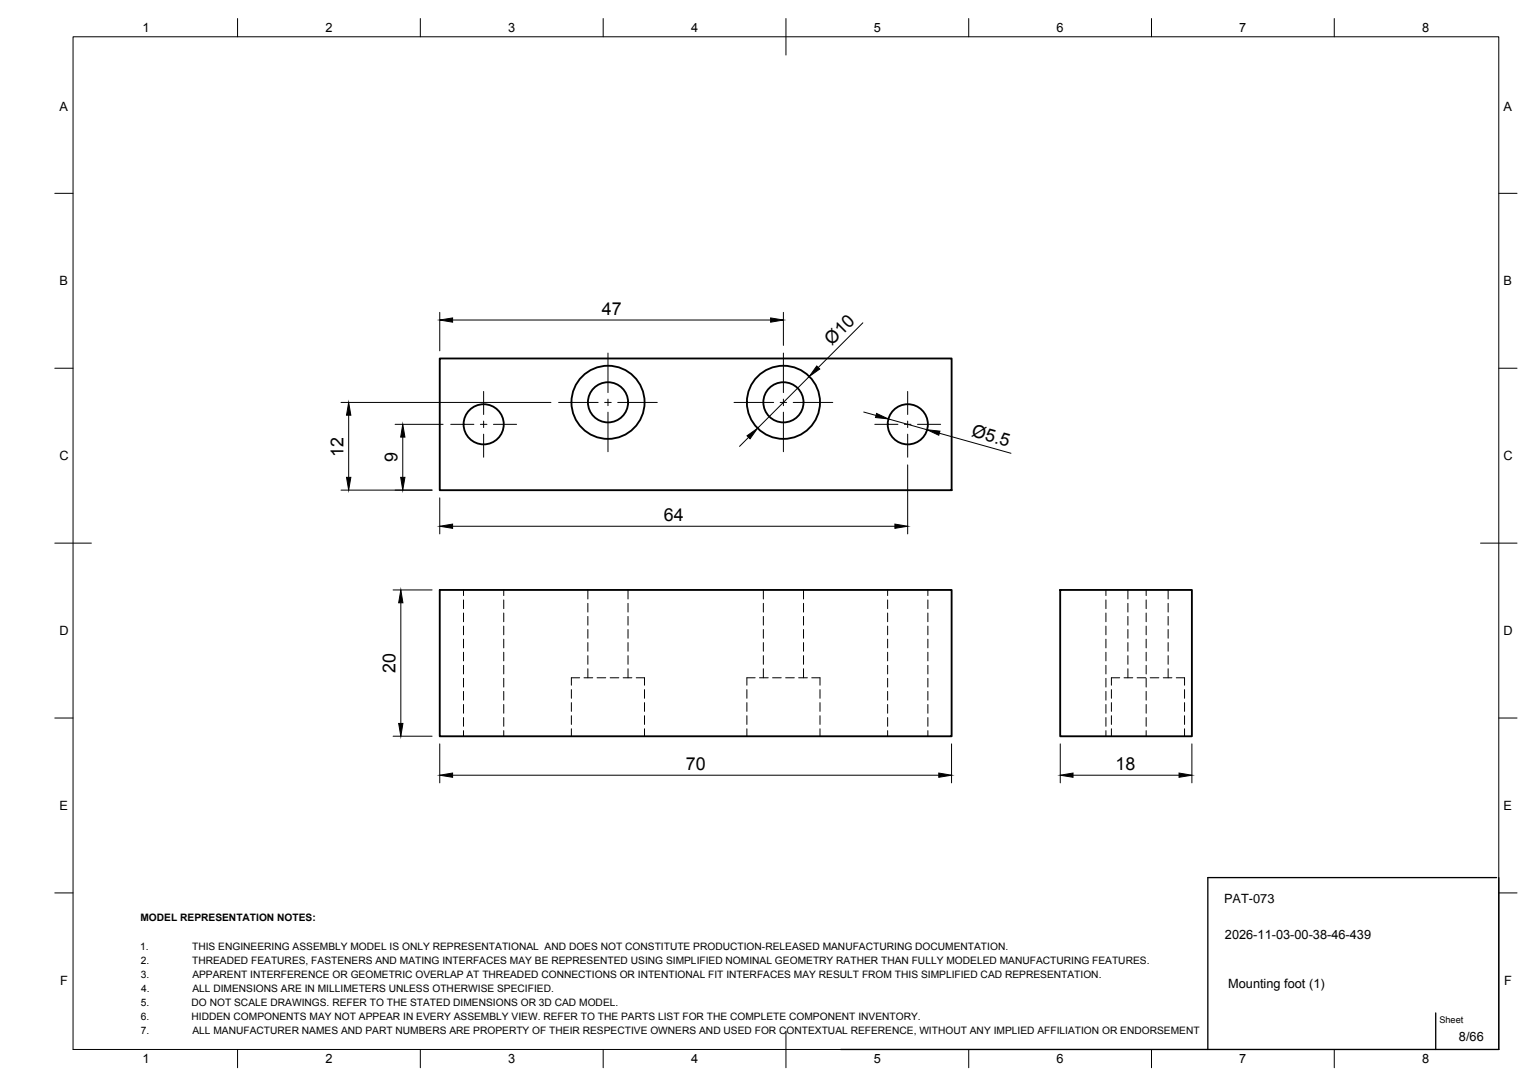
ISO-10303-21;
HEADER;
/* Generated by software containing ST-Developer
 * from STEP Tools, Inc. (www.steptools.com) 
 */

FILE_DESCRIPTION(
/* description */ ('Manual piston pump'),
/* implementation_level */ '2;1');

FILE_NAME(
/* name */ 'Mounting foot (1).step',
/* time_stamp */ '2026-11-02T16:54:23-08:00',
/* author */ (''),
/* organization */ (''),
/* preprocessor_version */ 'ST-DEVELOPER v20.2',
/* originating_system */ 'Autodesk Translation Framework v15.17.0.0',
/* authorisation */ '');

FILE_SCHEMA (('AUTOMOTIVE_DESIGN { 1 0 10303 214 3 1 1 }'));
ENDSEC;

DATA;
#10=MECHANICAL_DESIGN_GEOMETRIC_PRESENTATION_REPRESENTATION('',(#691),#19043);
#565=SHAPE_REPRESENTATION_RELATIONSHIP('SRR','None',#19311,#628);
#628=ADVANCED_BREP_SHAPE_REPRESENTATION('',(#763),#18978);
#691=STYLED_ITEM('',(#19662),#763);
#763=MANIFOLD_SOLID_BREP('Body1',#9475);
#864=FACE_BOUND('',#1974,.T.);
#865=FACE_BOUND('',#1977,.T.);
#866=FACE_BOUND('',#1985,.T.);
#867=FACE_BOUND('',#1986,.T.);
#868=FACE_BOUND('',#1987,.T.);
#869=FACE_BOUND('',#1988,.T.);
#870=FACE_BOUND('',#1990,.T.);
#871=FACE_BOUND('',#1991,.T.);
#872=FACE_BOUND('',#1992,.T.);
#873=FACE_BOUND('',#1993,.T.);
#1122=CYLINDRICAL_SURFACE('',#10379,0.275);
#1123=CYLINDRICAL_SURFACE('',#10382,0.275);
#1124=CYLINDRICAL_SURFACE('',#10385,0.5);
#1125=CYLINDRICAL_SURFACE('',#10390,0.5);
#1126=CYLINDRICAL_SURFACE('',#10395,0.275);
#1127=CYLINDRICAL_SURFACE('',#10397,0.275);
#1358=FACE_OUTER_BOUND('',#1970,.T.);
#1359=FACE_OUTER_BOUND('',#1971,.T.);
#1360=FACE_OUTER_BOUND('',#1972,.T.);
#1361=FACE_OUTER_BOUND('',#1973,.T.);
#1362=FACE_OUTER_BOUND('',#1975,.T.);
#1363=FACE_OUTER_BOUND('',#1976,.T.);
#1364=FACE_OUTER_BOUND('',#1978,.T.);
#1365=FACE_OUTER_BOUND('',#1979,.T.);
#1366=FACE_OUTER_BOUND('',#1980,.T.);
#1367=FACE_OUTER_BOUND('',#1981,.T.);
#1368=FACE_OUTER_BOUND('',#1982,.T.);
#1369=FACE_OUTER_BOUND('',#1983,.T.);
#1370=FACE_OUTER_BOUND('',#1984,.T.);
#1371=FACE_OUTER_BOUND('',#1989,.T.);
#1970=EDGE_LOOP('',(#6587,#6588,#6589,#6590));
#1971=EDGE_LOOP('',(#6591,#6592,#6593,#6594));
#1972=EDGE_LOOP('',(#6595,#6596,#6597,#6598));
#1973=EDGE_LOOP('',(#6599));
#1974=EDGE_LOOP('',(#6600));
#1975=EDGE_LOOP('',(#6601,#6602,#6603,#6604));
#1976=EDGE_LOOP('',(#6605));
#1977=EDGE_LOOP('',(#6606));
#1978=EDGE_LOOP('',(#6607,#6608,#6609,#6610));
#1979=EDGE_LOOP('',(#6611,#6612,#6613,#6614));
#1980=EDGE_LOOP('',(#6615,#6616,#6617,#6618));
#1981=EDGE_LOOP('',(#6619,#6620,#6621,#6622));
#1982=EDGE_LOOP('',(#6623,#6624,#6625,#6626));
#1983=EDGE_LOOP('',(#6627,#6628,#6629,#6630));
#1984=EDGE_LOOP('',(#6631,#6632,#6633,#6634));
#1985=EDGE_LOOP('',(#6635));
#1986=EDGE_LOOP('',(#6636));
#1987=EDGE_LOOP('',(#6637));
#1988=EDGE_LOOP('',(#6638));
#1989=EDGE_LOOP('',(#6639,#6640,#6641,#6642));
#1990=EDGE_LOOP('',(#6643));
#1991=EDGE_LOOP('',(#6644));
#1992=EDGE_LOOP('',(#6645));
#1993=EDGE_LOOP('',(#6646));
#2727=CIRCLE('',#10380,0.275);
#2728=CIRCLE('',#10381,0.275);
#2729=CIRCLE('',#10383,0.275);
#2730=CIRCLE('',#10384,0.275);
#2731=CIRCLE('',#10386,0.5);
#2732=CIRCLE('',#10387,0.5);
#2733=CIRCLE('',#10389,0.275);
#2734=CIRCLE('',#10391,0.5);
#2735=CIRCLE('',#10392,0.5);
#2736=CIRCLE('',#10394,0.275);
#2737=CIRCLE('',#10396,0.275);
#2738=CIRCLE('',#10398,0.275);
#3237=LINE('',#14991,#3841);
#3238=LINE('',#14997,#3842);
#3239=LINE('',#15003,#3843);
#3240=LINE('',#15012,#3844);
#3241=LINE('',#15019,#3845);
#3242=LINE('',#15023,#3846);
#3243=LINE('',#15028,#3847);
#3244=LINE('',#15030,#3848);
#3245=LINE('',#15032,#3849);
#3246=LINE('',#15033,#3850);
#3247=LINE('',#15036,#3851);
#3248=LINE('',#15038,#3852);
#3249=LINE('',#15039,#3853);
#3250=LINE('',#15042,#3854);
#3251=LINE('',#15044,#3855);
#3252=LINE('',#15045,#3856);
#3253=LINE('',#15047,#3857);
#3254=LINE('',#15048,#3858);
#3841=VECTOR('',#11861,0.275);
#3842=VECTOR('',#11868,0.275);
#3843=VECTOR('',#11875,0.5);
#3844=VECTOR('',#11886,0.5);
#3845=VECTOR('',#11895,0.275);
#3846=VECTOR('',#11900,0.275);
#3847=VECTOR('',#11905,1.);
#3848=VECTOR('',#11906,1.);
#3849=VECTOR('',#11907,1.);
#3850=VECTOR('',#11908,1.);
#3851=VECTOR('',#11911,1.);
#3852=VECTOR('',#11912,1.);
#3853=VECTOR('',#11913,1.);
#3854=VECTOR('',#11916,1.);
#3855=VECTOR('',#11917,1.);
#3856=VECTOR('',#11918,1.);
#3857=VECTOR('',#11921,1.);
#3858=VECTOR('',#11922,1.);
#4459=VERTEX_POINT('',#14988);
#4460=VERTEX_POINT('',#14990);
#4461=VERTEX_POINT('',#14994);
#4462=VERTEX_POINT('',#14996);
#4463=VERTEX_POINT('',#15000);
#4464=VERTEX_POINT('',#15002);
#4465=VERTEX_POINT('',#15006);
#4466=VERTEX_POINT('',#15009);
#4467=VERTEX_POINT('',#15011);
#4468=VERTEX_POINT('',#15015);
#4469=VERTEX_POINT('',#15018);
#4470=VERTEX_POINT('',#15022);
#4471=VERTEX_POINT('',#15026);
#4472=VERTEX_POINT('',#15027);
#4473=VERTEX_POINT('',#15029);
#4474=VERTEX_POINT('',#15031);
#4475=VERTEX_POINT('',#15035);
#4476=VERTEX_POINT('',#15037);
#4477=VERTEX_POINT('',#15041);
#4478=VERTEX_POINT('',#15043);
#5280=EDGE_CURVE('',#4459,#4459,#2727,.T.);
#5281=EDGE_CURVE('',#4459,#4460,#3237,.T.);
#5282=EDGE_CURVE('',#4460,#4460,#2728,.T.);
#5283=EDGE_CURVE('',#4461,#4461,#2729,.T.);
#5284=EDGE_CURVE('',#4461,#4462,#3238,.T.);
#5285=EDGE_CURVE('',#4462,#4462,#2730,.T.);
#5286=EDGE_CURVE('',#4463,#4463,#2731,.T.);
#5287=EDGE_CURVE('',#4463,#4464,#3239,.T.);
#5288=EDGE_CURVE('',#4464,#4464,#2732,.T.);
#5289=EDGE_CURVE('',#4465,#4465,#2733,.T.);
#5290=EDGE_CURVE('',#4466,#4466,#2734,.T.);
#5291=EDGE_CURVE('',#4466,#4467,#3240,.T.);
#5292=EDGE_CURVE('',#4467,#4467,#2735,.T.);
#5293=EDGE_CURVE('',#4468,#4468,#2736,.T.);
#5294=EDGE_CURVE('',#4465,#4469,#3241,.T.);
#5295=EDGE_CURVE('',#4469,#4469,#2737,.T.);
#5296=EDGE_CURVE('',#4468,#4470,#3242,.T.);
#5297=EDGE_CURVE('',#4470,#4470,#2738,.T.);
#5298=EDGE_CURVE('',#4471,#4472,#3243,.T.);
#5299=EDGE_CURVE('',#4472,#4473,#3244,.T.);
#5300=EDGE_CURVE('',#4474,#4473,#3245,.T.);
#5301=EDGE_CURVE('',#4471,#4474,#3246,.T.);
#5302=EDGE_CURVE('',#4475,#4471,#3247,.T.);
#5303=EDGE_CURVE('',#4476,#4474,#3248,.T.);
#5304=EDGE_CURVE('',#4475,#4476,#3249,.T.);
#5305=EDGE_CURVE('',#4477,#4475,#3250,.T.);
#5306=EDGE_CURVE('',#4478,#4476,#3251,.T.);
#5307=EDGE_CURVE('',#4477,#4478,#3252,.T.);
#5308=EDGE_CURVE('',#4472,#4477,#3253,.T.);
#5309=EDGE_CURVE('',#4473,#4478,#3254,.T.);
#6587=ORIENTED_EDGE('',*,*,#5280,.F.);
#6588=ORIENTED_EDGE('',*,*,#5281,.T.);
#6589=ORIENTED_EDGE('',*,*,#5282,.F.);
#6590=ORIENTED_EDGE('',*,*,#5281,.F.);
#6591=ORIENTED_EDGE('',*,*,#5283,.F.);
#6592=ORIENTED_EDGE('',*,*,#5284,.T.);
#6593=ORIENTED_EDGE('',*,*,#5285,.F.);
#6594=ORIENTED_EDGE('',*,*,#5284,.F.);
#6595=ORIENTED_EDGE('',*,*,#5286,.F.);
#6596=ORIENTED_EDGE('',*,*,#5287,.T.);
#6597=ORIENTED_EDGE('',*,*,#5288,.T.);
#6598=ORIENTED_EDGE('',*,*,#5287,.F.);
#6599=ORIENTED_EDGE('',*,*,#5288,.F.);
#6600=ORIENTED_EDGE('',*,*,#5289,.F.);
#6601=ORIENTED_EDGE('',*,*,#5290,.F.);
#6602=ORIENTED_EDGE('',*,*,#5291,.T.);
#6603=ORIENTED_EDGE('',*,*,#5292,.T.);
#6604=ORIENTED_EDGE('',*,*,#5291,.F.);
#6605=ORIENTED_EDGE('',*,*,#5292,.F.);
#6606=ORIENTED_EDGE('',*,*,#5293,.F.);
#6607=ORIENTED_EDGE('',*,*,#5289,.T.);
#6608=ORIENTED_EDGE('',*,*,#5294,.T.);
#6609=ORIENTED_EDGE('',*,*,#5295,.F.);
#6610=ORIENTED_EDGE('',*,*,#5294,.F.);
#6611=ORIENTED_EDGE('',*,*,#5293,.T.);
#6612=ORIENTED_EDGE('',*,*,#5296,.T.);
#6613=ORIENTED_EDGE('',*,*,#5297,.F.);
#6614=ORIENTED_EDGE('',*,*,#5296,.F.);
#6615=ORIENTED_EDGE('',*,*,#5298,.T.);
#6616=ORIENTED_EDGE('',*,*,#5299,.T.);
#6617=ORIENTED_EDGE('',*,*,#5300,.F.);
#6618=ORIENTED_EDGE('',*,*,#5301,.F.);
#6619=ORIENTED_EDGE('',*,*,#5302,.T.);
#6620=ORIENTED_EDGE('',*,*,#5301,.T.);
#6621=ORIENTED_EDGE('',*,*,#5303,.F.);
#6622=ORIENTED_EDGE('',*,*,#5304,.F.);
#6623=ORIENTED_EDGE('',*,*,#5305,.T.);
#6624=ORIENTED_EDGE('',*,*,#5304,.T.);
#6625=ORIENTED_EDGE('',*,*,#5306,.F.);
#6626=ORIENTED_EDGE('',*,*,#5307,.F.);
#6627=ORIENTED_EDGE('',*,*,#5308,.T.);
#6628=ORIENTED_EDGE('',*,*,#5307,.T.);
#6629=ORIENTED_EDGE('',*,*,#5309,.F.);
#6630=ORIENTED_EDGE('',*,*,#5299,.F.);
#6631=ORIENTED_EDGE('',*,*,#5309,.T.);
#6632=ORIENTED_EDGE('',*,*,#5306,.T.);
#6633=ORIENTED_EDGE('',*,*,#5303,.T.);
#6634=ORIENTED_EDGE('',*,*,#5300,.T.);
#6635=ORIENTED_EDGE('',*,*,#5282,.T.);
#6636=ORIENTED_EDGE('',*,*,#5285,.T.);
#6637=ORIENTED_EDGE('',*,*,#5295,.T.);
#6638=ORIENTED_EDGE('',*,*,#5297,.T.);
#6639=ORIENTED_EDGE('',*,*,#5308,.F.);
#6640=ORIENTED_EDGE('',*,*,#5298,.F.);
#6641=ORIENTED_EDGE('',*,*,#5302,.F.);
#6642=ORIENTED_EDGE('',*,*,#5305,.F.);
#6643=ORIENTED_EDGE('',*,*,#5280,.T.);
#6644=ORIENTED_EDGE('',*,*,#5283,.T.);
#6645=ORIENTED_EDGE('',*,*,#5286,.T.);
#6646=ORIENTED_EDGE('',*,*,#5290,.T.);
#8608=PLANE('',#10388);
#8609=PLANE('',#10393);
#8610=PLANE('',#10399);
#8611=PLANE('',#10400);
#8612=PLANE('',#10401);
#8613=PLANE('',#10402);
#8614=PLANE('',#10403);
#8615=PLANE('',#10404);
#8963=ADVANCED_FACE('',(#1358),#1122,.F.);
#8964=ADVANCED_FACE('',(#1359),#1123,.F.);
#8965=ADVANCED_FACE('',(#1360),#1124,.F.);
#8966=ADVANCED_FACE('',(#1361,#864),#8608,.F.);
#8967=ADVANCED_FACE('',(#1362),#1125,.F.);
#8968=ADVANCED_FACE('',(#1363,#865),#8609,.F.);
#8969=ADVANCED_FACE('',(#1364),#1126,.F.);
#8970=ADVANCED_FACE('',(#1365),#1127,.F.);
#8971=ADVANCED_FACE('',(#1366),#8610,.T.);
#8972=ADVANCED_FACE('',(#1367),#8611,.T.);
#8973=ADVANCED_FACE('',(#1368),#8612,.T.);
#8974=ADVANCED_FACE('',(#1369),#8613,.T.);
#8975=ADVANCED_FACE('',(#1370,#866,#867,#868,#869),#8614,.T.);
#8976=ADVANCED_FACE('',(#1371,#870,#871,#872,#873),#8615,.F.);
#9475=CLOSED_SHELL('',(#8963,#8964,#8965,#8966,#8967,#8968,#8969,#8970,
#8971,#8972,#8973,#8974,#8975,#8976));
#10378=AXIS2_PLACEMENT_3D('',#14986,#11855,#11856);
#10379=AXIS2_PLACEMENT_3D('',#14987,#11857,#11858);
#10380=AXIS2_PLACEMENT_3D('',#14989,#11859,#11860);
#10381=AXIS2_PLACEMENT_3D('',#14992,#11862,#11863);
#10382=AXIS2_PLACEMENT_3D('',#14993,#11864,#11865);
#10383=AXIS2_PLACEMENT_3D('',#14995,#11866,#11867);
#10384=AXIS2_PLACEMENT_3D('',#14998,#11869,#11870);
#10385=AXIS2_PLACEMENT_3D('',#14999,#11871,#11872);
#10386=AXIS2_PLACEMENT_3D('',#15001,#11873,#11874);
#10387=AXIS2_PLACEMENT_3D('',#15004,#11876,#11877);
#10388=AXIS2_PLACEMENT_3D('',#15005,#11878,#11879);
#10389=AXIS2_PLACEMENT_3D('',#15007,#11880,#11881);
#10390=AXIS2_PLACEMENT_3D('',#15008,#11882,#11883);
#10391=AXIS2_PLACEMENT_3D('',#15010,#11884,#11885);
#10392=AXIS2_PLACEMENT_3D('',#15013,#11887,#11888);
#10393=AXIS2_PLACEMENT_3D('',#15014,#11889,#11890);
#10394=AXIS2_PLACEMENT_3D('',#15016,#11891,#11892);
#10395=AXIS2_PLACEMENT_3D('',#15017,#11893,#11894);
#10396=AXIS2_PLACEMENT_3D('',#15020,#11896,#11897);
#10397=AXIS2_PLACEMENT_3D('',#15021,#11898,#11899);
#10398=AXIS2_PLACEMENT_3D('',#15024,#11901,#11902);
#10399=AXIS2_PLACEMENT_3D('',#15025,#11903,#11904);
#10400=AXIS2_PLACEMENT_3D('',#15034,#11909,#11910);
#10401=AXIS2_PLACEMENT_3D('',#15040,#11914,#11915);
#10402=AXIS2_PLACEMENT_3D('',#15046,#11919,#11920);
#10403=AXIS2_PLACEMENT_3D('',#15049,#11923,#11924);
#10404=AXIS2_PLACEMENT_3D('',#15050,#11925,#11926);
#11855=DIRECTION('axis',(0.,0.,1.));
#11856=DIRECTION('refdir',(1.,0.,0.));
#11857=DIRECTION('center_axis',(0.,0.,1.));
#11858=DIRECTION('ref_axis',(1.,0.,0.));
#11859=DIRECTION('center_axis',(0.,0.,1.));
#11860=DIRECTION('ref_axis',(1.,0.,0.));
#11861=DIRECTION('',(0.,0.,1.));
#11862=DIRECTION('center_axis',(0.,0.,-1.));
#11863=DIRECTION('ref_axis',(1.,0.,0.));
#11864=DIRECTION('center_axis',(0.,0.,1.));
#11865=DIRECTION('ref_axis',(1.,0.,0.));
#11866=DIRECTION('center_axis',(0.,0.,1.));
#11867=DIRECTION('ref_axis',(1.,0.,0.));
#11868=DIRECTION('',(0.,0.,1.));
#11869=DIRECTION('center_axis',(0.,0.,-1.));
#11870=DIRECTION('ref_axis',(1.,0.,0.));
#11871=DIRECTION('center_axis',(0.,0.,1.));
#11872=DIRECTION('ref_axis',(1.,0.,0.));
#11873=DIRECTION('center_axis',(0.,0.,1.));
#11874=DIRECTION('ref_axis',(1.,0.,0.));
#11875=DIRECTION('',(0.,0.,1.));
#11876=DIRECTION('center_axis',(0.,0.,1.));
#11877=DIRECTION('ref_axis',(1.,0.,0.));
#11878=DIRECTION('center_axis',(0.,0.,1.));
#11879=DIRECTION('ref_axis',(1.,0.,0.));
#11880=DIRECTION('center_axis',(0.,0.,-1.));
#11881=DIRECTION('ref_axis',(1.,0.,0.));
#11882=DIRECTION('center_axis',(0.,0.,1.));
#11883=DIRECTION('ref_axis',(1.,0.,0.));
#11884=DIRECTION('center_axis',(0.,0.,1.));
#11885=DIRECTION('ref_axis',(1.,0.,0.));
#11886=DIRECTION('',(0.,0.,1.));
#11887=DIRECTION('center_axis',(0.,0.,1.));
#11888=DIRECTION('ref_axis',(1.,0.,0.));
#11889=DIRECTION('center_axis',(0.,0.,1.));
#11890=DIRECTION('ref_axis',(1.,0.,0.));
#11891=DIRECTION('center_axis',(0.,0.,-1.));
#11892=DIRECTION('ref_axis',(1.,0.,0.));
#11893=DIRECTION('center_axis',(0.,0.,1.));
#11894=DIRECTION('ref_axis',(1.,0.,0.));
#11895=DIRECTION('',(0.,0.,1.));
#11896=DIRECTION('center_axis',(0.,0.,-1.));
#11897=DIRECTION('ref_axis',(1.,0.,0.));
#11898=DIRECTION('center_axis',(0.,0.,1.));
#11899=DIRECTION('ref_axis',(1.,0.,0.));
#11900=DIRECTION('',(0.,0.,1.));
#11901=DIRECTION('center_axis',(0.,0.,-1.));
#11902=DIRECTION('ref_axis',(1.,0.,0.));
#11903=DIRECTION('center_axis',(0.,1.,0.));
#11904=DIRECTION('ref_axis',(-1.,0.,0.));
#11905=DIRECTION('',(-1.,0.,0.));
#11906=DIRECTION('',(0.,0.,1.));
#11907=DIRECTION('',(-1.,0.,0.));
#11908=DIRECTION('',(0.,0.,1.));
#11909=DIRECTION('center_axis',(1.,0.,0.));
#11910=DIRECTION('ref_axis',(0.,1.,0.));
#11911=DIRECTION('',(0.,1.,0.));
#11912=DIRECTION('',(0.,1.,0.));
#11913=DIRECTION('',(0.,0.,1.));
#11914=DIRECTION('center_axis',(0.,-1.,0.));
#11915=DIRECTION('ref_axis',(1.,0.,0.));
#11916=DIRECTION('',(1.,0.,0.));
#11917=DIRECTION('',(1.,0.,0.));
#11918=DIRECTION('',(0.,0.,1.));
#11919=DIRECTION('center_axis',(-1.,0.,0.));
#11920=DIRECTION('ref_axis',(0.,-1.,0.));
#11921=DIRECTION('',(0.,-1.,0.));
#11922=DIRECTION('',(0.,-1.,0.));
#11923=DIRECTION('center_axis',(0.,0.,1.));
#11924=DIRECTION('ref_axis',(1.,0.,0.));
#11925=DIRECTION('center_axis',(0.,0.,1.));
#11926=DIRECTION('ref_axis',(1.,0.,0.));
#14986=CARTESIAN_POINT('',(0.,0.,0.));
#14987=CARTESIAN_POINT('Origin',(-2.9,11.7,-0.1));
#14988=CARTESIAN_POINT('',(-3.175,11.7,0.));
#14989=CARTESIAN_POINT('Origin',(-2.9,11.7,0.));
#14990=CARTESIAN_POINT('',(-3.175,11.7,2.));
#14991=CARTESIAN_POINT('',(-3.175,11.7,-0.1));
#14992=CARTESIAN_POINT('Origin',(-2.9,11.7,2.));
#14993=CARTESIAN_POINT('Origin',(2.9,11.7,-0.1));
#14994=CARTESIAN_POINT('',(2.625,11.7,0.));
#14995=CARTESIAN_POINT('Origin',(2.9,11.7,0.));
#14996=CARTESIAN_POINT('',(2.625,11.7,2.));
#14997=CARTESIAN_POINT('',(2.625,11.7,-0.1));
#14998=CARTESIAN_POINT('Origin',(2.9,11.7,2.));
#14999=CARTESIAN_POINT('Origin',(-1.2,12.,-0.1));
#15000=CARTESIAN_POINT('',(-1.7,12.,0.));
#15001=CARTESIAN_POINT('Origin',(-1.2,12.,0.));
#15002=CARTESIAN_POINT('',(-1.7,12.,0.8));
#15003=CARTESIAN_POINT('',(-1.7,12.,-0.1));
#15004=CARTESIAN_POINT('Origin',(-1.2,12.,0.8));
#15005=CARTESIAN_POINT('Origin',(-1.2,12.,0.8));
#15006=CARTESIAN_POINT('',(-1.475,12.,0.8));
#15007=CARTESIAN_POINT('Origin',(-1.2,12.,0.8));
#15008=CARTESIAN_POINT('Origin',(1.2,12.,-0.1));
#15009=CARTESIAN_POINT('',(0.7,12.,0.));
#15010=CARTESIAN_POINT('Origin',(1.2,12.,0.));
#15011=CARTESIAN_POINT('',(0.7,12.,0.8));
#15012=CARTESIAN_POINT('',(0.7,12.,-0.1));
#15013=CARTESIAN_POINT('Origin',(1.2,12.,0.8));
#15014=CARTESIAN_POINT('Origin',(1.2,12.,0.8));
#15015=CARTESIAN_POINT('',(0.925,12.,0.8));
#15016=CARTESIAN_POINT('Origin',(1.2,12.,0.8));
#15017=CARTESIAN_POINT('Origin',(-1.2,12.,-0.1));
#15018=CARTESIAN_POINT('',(-1.475,12.,2.));
#15019=CARTESIAN_POINT('',(-1.475,12.,-0.1));
#15020=CARTESIAN_POINT('Origin',(-1.2,12.,2.));
#15021=CARTESIAN_POINT('Origin',(1.2,12.,-0.1));
#15022=CARTESIAN_POINT('',(0.925,12.,2.));
#15023=CARTESIAN_POINT('',(0.925,12.,-0.1));
#15024=CARTESIAN_POINT('Origin',(1.2,12.,2.));
#15025=CARTESIAN_POINT('Origin',(3.5,12.6,0.));
#15026=CARTESIAN_POINT('',(3.5,12.6,0.));
#15027=CARTESIAN_POINT('',(-3.5,12.6,0.));
#15028=CARTESIAN_POINT('',(3.5,12.6,0.));
#15029=CARTESIAN_POINT('',(-3.5,12.6,2.));
#15030=CARTESIAN_POINT('',(-3.5,12.6,0.));
#15031=CARTESIAN_POINT('',(3.5,12.6,2.));
#15032=CARTESIAN_POINT('',(3.5,12.6,2.));
#15033=CARTESIAN_POINT('',(3.5,12.6,0.));
#15034=CARTESIAN_POINT('Origin',(3.5,10.8,0.));
#15035=CARTESIAN_POINT('',(3.5,10.8,0.));
#15036=CARTESIAN_POINT('',(3.5,10.8,0.));
#15037=CARTESIAN_POINT('',(3.5,10.8,2.));
#15038=CARTESIAN_POINT('',(3.5,10.8,2.));
#15039=CARTESIAN_POINT('',(3.5,10.8,0.));
#15040=CARTESIAN_POINT('Origin',(-3.5,10.8,0.));
#15041=CARTESIAN_POINT('',(-3.5,10.8,0.));
#15042=CARTESIAN_POINT('',(-3.5,10.8,0.));
#15043=CARTESIAN_POINT('',(-3.5,10.8,2.));
#15044=CARTESIAN_POINT('',(-3.5,10.8,2.));
#15045=CARTESIAN_POINT('',(-3.5,10.8,0.));
#15046=CARTESIAN_POINT('Origin',(-3.5,12.6,0.));
#15047=CARTESIAN_POINT('',(-3.5,12.6,0.));
#15048=CARTESIAN_POINT('',(-3.5,12.6,2.));
#15049=CARTESIAN_POINT('Origin',(0.,11.7,2.));
#15050=CARTESIAN_POINT('Origin',(0.,11.7,0.));
#18907=UNCERTAINTY_MEASURE_WITH_UNIT(LENGTH_MEASURE(0.001),#19044,
'DISTANCE_ACCURACY_VALUE',
'Maximum model space distance between geometric entities at asserted c
onnectivities');
#18972=UNCERTAINTY_MEASURE_WITH_UNIT(LENGTH_MEASURE(0.001),#19044,
'DISTANCE_ACCURACY_VALUE',
'Maximum model space distance between geometric entities at asserted c
onnectivities');
#18978=(
GEOMETRIC_REPRESENTATION_CONTEXT(3)
GLOBAL_UNCERTAINTY_ASSIGNED_CONTEXT((#18907))
GLOBAL_UNIT_ASSIGNED_CONTEXT((#19044,#19046,#19047))
REPRESENTATION_CONTEXT('','3D')
);
#19043=(
GEOMETRIC_REPRESENTATION_CONTEXT(3)
GLOBAL_UNCERTAINTY_ASSIGNED_CONTEXT((#18972))
GLOBAL_UNIT_ASSIGNED_CONTEXT((#19044,#19046,#19047))
REPRESENTATION_CONTEXT('','3D')
);
#19044=(
LENGTH_UNIT()
NAMED_UNIT(*)
SI_UNIT(.CENTI.,.METRE.)
);
#19046=(
NAMED_UNIT(*)
PLANE_ANGLE_UNIT()
SI_UNIT($,.RADIAN.)
);
#19047=(
NAMED_UNIT(*)
SI_UNIT($,.STERADIAN.)
SOLID_ANGLE_UNIT()
);
#19053=SHAPE_DEFINITION_REPRESENTATION(#19123,#19311);
#19123=PRODUCT_DEFINITION_SHAPE('',$,#19382);
#19311=SHAPE_REPRESENTATION('',(#10378),#18978);
#19376=PRODUCT_DEFINITION_CONTEXT('part definition',#19588,'design');
#19382=PRODUCT_DEFINITION('2026-11-03-00-38-46-439','Mounting foot (1)',
#19452,#19376);
#19452=PRODUCT_DEFINITION_FORMATION('',$,#19595);
#19588=APPLICATION_CONTEXT(
'Core Data for Automotive Mechanical Design Process');
#19589=PRODUCT_CONTEXT('part definition',#19588,'mechanical');
#19595=PRODUCT('2026-11-03-00-38-46-439','Mounting foot (1)',
'Mounting foot',(#19589));
#19662=PRESENTATION_STYLE_ASSIGNMENT((#19668));
#19668=SURFACE_STYLE_USAGE(.BOTH.,#19674);
#19674=SURFACE_SIDE_STYLE('',(#19680));
#19680=SURFACE_STYLE_FILL_AREA(#19686);
#19686=FILL_AREA_STYLE('CAD Library Painted - Deep blue',(#19692));
#19692=FILL_AREA_STYLE_COLOUR('CAD Library Painted - Deep blue',#19698);
#19698=COLOUR_RGB('CAD Library Painted - Deep blue',0.0784313725490196,
0.203921568627451,0.349019607843137);
ENDSEC;
END-ISO-10303-21;
